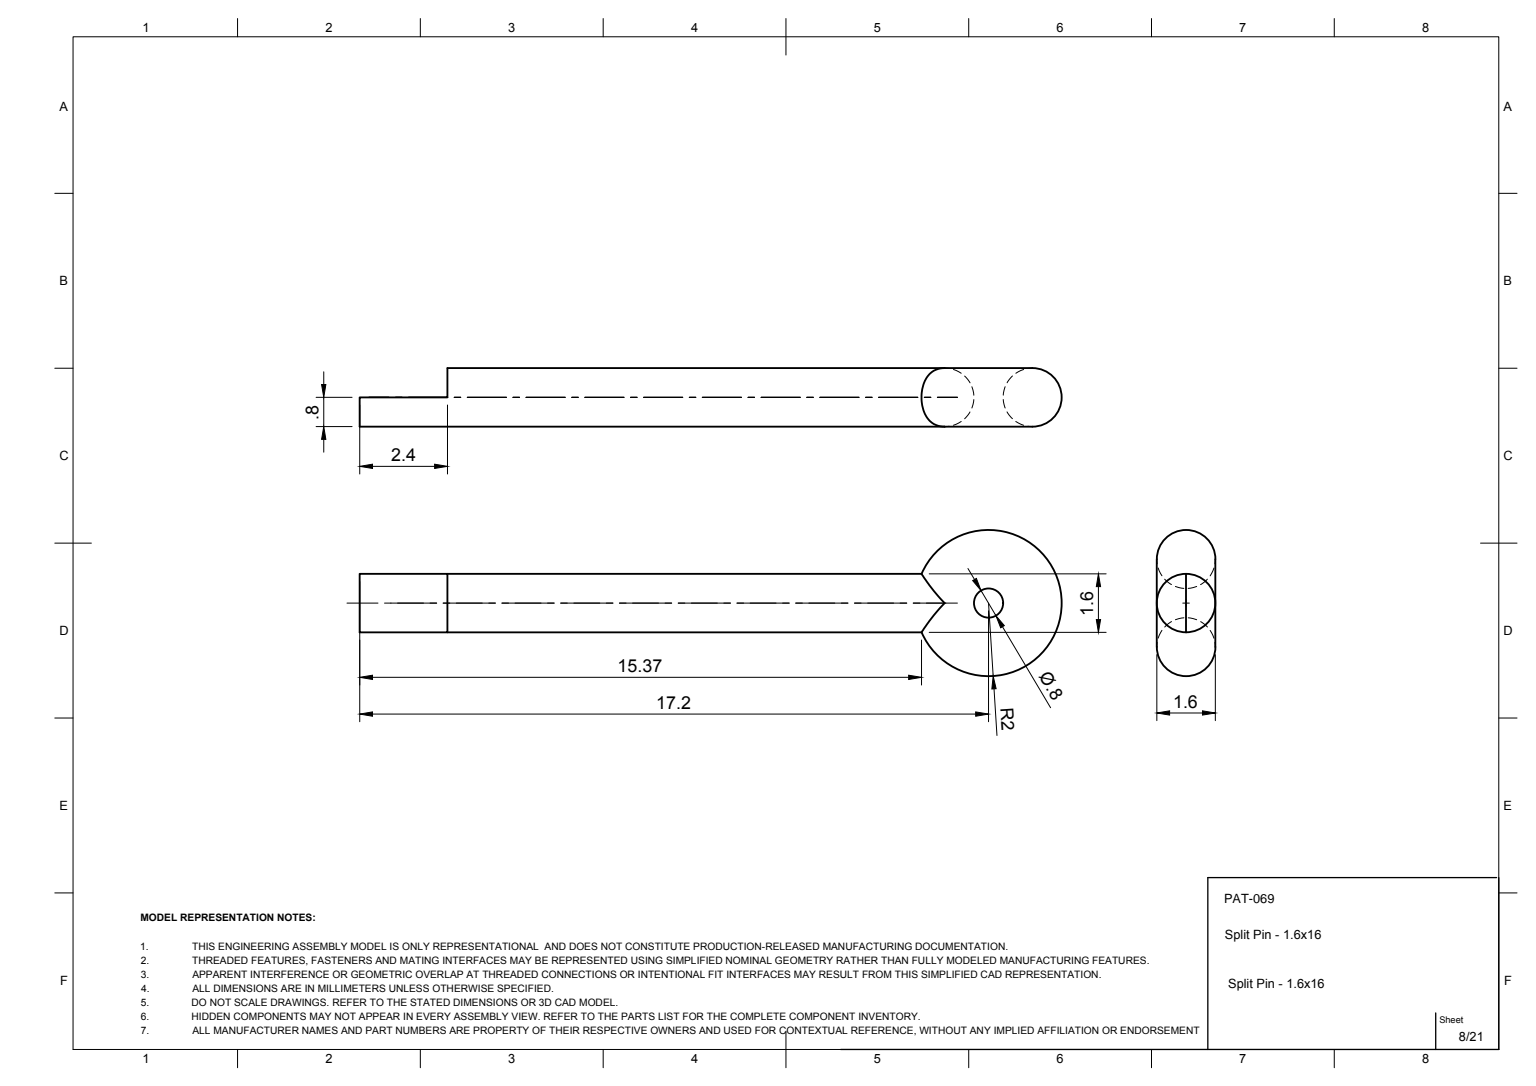
ISO-10303-21;
HEADER;
/* Generated by software containing ST-Developer
 * from STEP Tools, Inc. (www.steptools.com) 
 */

FILE_DESCRIPTION(
/* description */ ('Located fixture plate with toggle clamp'),
/* implementation_level */ '2;1');

FILE_NAME(
/* name */ 'Split Pin - 1.6x16.step',
/* time_stamp */ '2026-10-27T21:36:12-07:00',
/* author */ (''),
/* organization */ (''),
/* preprocessor_version */ 'ST-DEVELOPER v20.2',
/* originating_system */ 'Autodesk Translation Framework v15.17.0.0',
/* authorisation */ '');

FILE_SCHEMA (('AUTOMOTIVE_DESIGN { 1 0 10303 214 3 1 1 }'));
ENDSEC;

DATA;
#10=MECHANICAL_DESIGN_GEOMETRIC_PRESENTATION_REPRESENTATION('',(#344),#9285);
#11=TOROIDAL_SURFACE('',#5974,0.12,0.08);
#16=B_SPLINE_CURVE_WITH_KNOTS('',3,(#9112,#9113,#9114,#9115,#9116,#9117,
#9118,#9119,#9120,#9121,#9122,#9123,#9124,#9125,#9126,#9127,#9128,#9129,
#9130,#9131,#9132,#9133,#9134,#9135,#9136,#9137),.UNSPECIFIED.,.F.,.F.,
(4,2,2,2,2,2,2,2,2,2,2,2,4),(-0.00054581412719389,0.,0.0281583564005144,
0.0618496465371181,0.0905865724114538,0.120694112793616,0.144966158459363,
0.16923820412511,0.199345744507272,0.228082670381608,0.261773960518212,
0.289932316918681,0.290478131045882),.UNSPECIFIED.);
#17=B_SPLINE_CURVE_WITH_KNOTS('',3,(#9138,#9139,#9140,#9141,#9142,#9143,
#9144,#9145,#9146,#9147,#9148,#9149,#9150,#9151,#9152,#9153,#9154,#9155,
#9156,#9157,#9158,#9159,#9160,#9161,#9162,#9163),.UNSPECIFIED.,.F.,.F.,
(4,2,2,2,2,2,2,2,2,2,2,2,4),(-0.000545814127196571,0.,0.0281583564006391,
0.0618496465374156,0.0905865724118984,0.120694112794215,0.144966158460086,
0.169238204125958,0.199345744508275,0.228082670382758,0.261773960519534,
0.289932316920171,0.29047813104737),.UNSPECIFIED.);
#296=SHAPE_REPRESENTATION_RELATIONSHIP('SRR','None',#9422,#320);
#320=ADVANCED_BREP_SHAPE_REPRESENTATION('',(#365),#9284);
#344=STYLED_ITEM('',(#9612),#365);
#365=MANIFOLD_SOLID_BREP('Body1',#5195);
#485=FACE_BOUND('',#1378,.T.);
#670=PLANE('',#5977);
#671=PLANE('',#5979);
#672=PLANE('',#5983);
#963=FACE_OUTER_BOUND('',#1377,.T.);
#964=FACE_OUTER_BOUND('',#1379,.T.);
#965=FACE_OUTER_BOUND('',#1380,.T.);
#966=FACE_OUTER_BOUND('',#1381,.T.);
#967=FACE_OUTER_BOUND('',#1382,.T.);
#1377=EDGE_LOOP('',(#4768,#4769,#4770,#4771));
#1378=EDGE_LOOP('',(#4772,#4773));
#1379=EDGE_LOOP('',(#4774,#4775));
#1380=EDGE_LOOP('',(#4776,#4777,#4778,#4779));
#1381=EDGE_LOOP('',(#4780,#4781,#4782,#4783,#4784,#4785,#4786,#4787,#4788));
#1382=EDGE_LOOP('',(#4789,#4790,#4791));
#1576=CIRCLE('',#5975,0.08);
#1577=CIRCLE('',#5976,0.04);
#1578=CIRCLE('',#5978,0.08);
#1579=CIRCLE('',#5981,0.08);
#1580=CIRCLE('',#5982,0.08);
#1986=LINE('',#9168,#2396);
#1987=LINE('',#9171,#2397);
#1988=LINE('',#9173,#2398);
#1989=LINE('',#9174,#2399);
#1990=LINE('',#9178,#2400);
#2396=VECTOR('',#7470,1.);
#2397=VECTOR('',#7473,1.);
#2398=VECTOR('',#7474,1.);
#2399=VECTOR('',#7475,1.);
#2400=VECTOR('',#7480,0.08);
#2822=VERTEX_POINT('',#9107);
#2823=VERTEX_POINT('',#9110);
#2824=VERTEX_POINT('',#9111);
#2825=VERTEX_POINT('',#9165);
#2826=VERTEX_POINT('',#9166);
#2827=VERTEX_POINT('',#9170);
#2828=VERTEX_POINT('',#9172);
#2829=VERTEX_POINT('',#9176);
#3472=EDGE_CURVE('',#2822,#2822,#1576,.T.);
#3473=EDGE_CURVE('',#2822,#2822,#1577,.T.);
#3474=EDGE_CURVE('',#2823,#2824,#16,.T.);
#3475=EDGE_CURVE('',#2824,#2823,#17,.T.);
#3476=EDGE_CURVE('',#2825,#2826,#1578,.T.);
#3477=EDGE_CURVE('',#2825,#2826,#1986,.T.);
#3478=EDGE_CURVE('',#2826,#2827,#1987,.T.);
#3479=EDGE_CURVE('',#2828,#2827,#1988,.T.);
#3480=EDGE_CURVE('',#2825,#2828,#1989,.T.);
#3481=EDGE_CURVE('',#2829,#2828,#1579,.T.);
#3482=EDGE_CURVE('',#2829,#2824,#1990,.T.);
#3483=EDGE_CURVE('',#2827,#2829,#1580,.T.);
#4768=ORIENTED_EDGE('',*,*,#3472,.F.);
#4769=ORIENTED_EDGE('',*,*,#3473,.T.);
#4770=ORIENTED_EDGE('',*,*,#3472,.T.);
#4771=ORIENTED_EDGE('',*,*,#3473,.F.);
#4772=ORIENTED_EDGE('',*,*,#3474,.F.);
#4773=ORIENTED_EDGE('',*,*,#3475,.F.);
#4774=ORIENTED_EDGE('',*,*,#3476,.T.);
#4775=ORIENTED_EDGE('',*,*,#3477,.F.);
#4776=ORIENTED_EDGE('',*,*,#3477,.T.);
#4777=ORIENTED_EDGE('',*,*,#3478,.T.);
#4778=ORIENTED_EDGE('',*,*,#3479,.F.);
#4779=ORIENTED_EDGE('',*,*,#3480,.F.);
#4780=ORIENTED_EDGE('',*,*,#3476,.F.);
#4781=ORIENTED_EDGE('',*,*,#3480,.T.);
#4782=ORIENTED_EDGE('',*,*,#3481,.F.);
#4783=ORIENTED_EDGE('',*,*,#3482,.T.);
#4784=ORIENTED_EDGE('',*,*,#3475,.T.);
#4785=ORIENTED_EDGE('',*,*,#3474,.T.);
#4786=ORIENTED_EDGE('',*,*,#3482,.F.);
#4787=ORIENTED_EDGE('',*,*,#3483,.F.);
#4788=ORIENTED_EDGE('',*,*,#3478,.F.);
#4789=ORIENTED_EDGE('',*,*,#3483,.T.);
#4790=ORIENTED_EDGE('',*,*,#3481,.T.);
#4791=ORIENTED_EDGE('',*,*,#3479,.T.);
#4873=CYLINDRICAL_SURFACE('',#5980,0.08);
#5164=ADVANCED_FACE('',(#963,#485),#11,.T.);
#5165=ADVANCED_FACE('',(#964),#670,.F.);
#5166=ADVANCED_FACE('',(#965),#671,.T.);
#5167=ADVANCED_FACE('',(#966),#4873,.T.);
#5168=ADVANCED_FACE('',(#967),#672,.F.);
#5195=CLOSED_SHELL('',(#5164,#5165,#5166,#5167,#5168));
#5973=AXIS2_PLACEMENT_3D('',#9105,#7458,#7459);
#5974=AXIS2_PLACEMENT_3D('',#9106,#7460,#7461);
#5975=AXIS2_PLACEMENT_3D('',#9108,#7462,#7463);
#5976=AXIS2_PLACEMENT_3D('',#9109,#7464,#7465);
#5977=AXIS2_PLACEMENT_3D('',#9164,#7466,#7467);
#5978=AXIS2_PLACEMENT_3D('',#9167,#7468,#7469);
#5979=AXIS2_PLACEMENT_3D('',#9169,#7471,#7472);
#5980=AXIS2_PLACEMENT_3D('',#9175,#7476,#7477);
#5981=AXIS2_PLACEMENT_3D('',#9177,#7478,#7479);
#5982=AXIS2_PLACEMENT_3D('',#9179,#7481,#7482);
#5983=AXIS2_PLACEMENT_3D('',#9180,#7483,#7484);
#7458=DIRECTION('axis',(0.,0.,1.));
#7459=DIRECTION('refdir',(1.,0.,0.));
#7460=DIRECTION('center_axis',(-1.,0.,0.));
#7461=DIRECTION('ref_axis',(0.,0.,1.));
#7462=DIRECTION('center_axis',(0.,-1.,1.38777878078145E-16));
#7463=DIRECTION('ref_axis',(0.,-1.38777878078145E-16,-1.));
#7464=DIRECTION('center_axis',(1.,0.,0.));
#7465=DIRECTION('ref_axis',(0.,0.,1.));
#7466=DIRECTION('center_axis',(0.,1.,0.));
#7467=DIRECTION('ref_axis',(1.,0.,0.));
#7468=DIRECTION('center_axis',(0.,-1.,0.));
#7469=DIRECTION('ref_axis',(1.,0.,0.));
#7470=DIRECTION('',(0.,0.,1.));
#7471=DIRECTION('center_axis',(1.,0.,0.));
#7472=DIRECTION('ref_axis',(0.,0.,1.));
#7473=DIRECTION('',(0.,-1.,0.));
#7474=DIRECTION('',(0.,0.,1.));
#7475=DIRECTION('',(0.,-1.,0.));
#7476=DIRECTION('center_axis',(0.,-1.,0.));
#7477=DIRECTION('ref_axis',(1.,0.,0.));
#7478=DIRECTION('center_axis',(0.,-1.,0.));
#7479=DIRECTION('ref_axis',(1.,0.,0.));
#7480=DIRECTION('',(0.,1.,0.));
#7481=DIRECTION('center_axis',(0.,-1.,0.));
#7482=DIRECTION('ref_axis',(1.,0.,0.));
#7483=DIRECTION('center_axis',(0.,1.,0.));
#7484=DIRECTION('ref_axis',(1.,0.,0.));
#9105=CARTESIAN_POINT('',(0.,0.,0.));
#9106=CARTESIAN_POINT('Origin',(0.,0.12,0.));
#9107=CARTESIAN_POINT('',(-9.79717439317883E-18,0.12,-0.04));
#9108=CARTESIAN_POINT('Origin',(0.,0.12,-0.12));
#9109=CARTESIAN_POINT('Origin',(9.79717439317883E-18,0.12,0.));
#9110=CARTESIAN_POINT('',(0.08,-4.89858719658941E-18,7.34788079488412E-18));
#9111=CARTESIAN_POINT('',(-0.08,-4.89858719658941E-18,7.34788079488412E-18));
#9112=CARTESIAN_POINT('Ctrl Pts',(0.08,-4.89858719658941E-18,7.34788079488412E-18));
#9113=CARTESIAN_POINT('Ctrl Pts',(0.08,-0.00012864962353541,0.000128649623535413));
#9114=CARTESIAN_POINT('Ctrl Pts',(0.0799996896739287,-0.00025719571182076,
0.000257402596003253));
#9115=CARTESIAN_POINT('Ctrl Pts',(0.0799669711262291,-0.00701193164572964,
0.00703384588894362));
#9116=CARTESIAN_POINT('Ctrl Pts',(0.0791054994909294,-0.0133457972655825,
0.0139383126556792));
#9117=CARTESIAN_POINT('Ctrl Pts',(0.0749700088488058,-0.0265076530862524,
0.0292212026164895));
#9118=CARTESIAN_POINT('Ctrl Pts',(0.0712702072865517,-0.0331317062461458,
0.0375603420117568));
#9119=CARTESIAN_POINT('Ctrl Pts',(0.0612858949407667,-0.0440683985740427,
0.0520545604187517));
#9120=CARTESIAN_POINT('Ctrl Pts',(0.0555090276731744,-0.0485199197794574,
0.0582717815295611));
#9121=CARTESIAN_POINT('Ctrl Pts',(0.0412398082144208,-0.0561090538733877,
0.0691638397919718));
#9122=CARTESIAN_POINT('Ctrl Pts',(0.0327878980890048,-0.059089642483296,
0.0736229049587921));
#9123=CARTESIAN_POINT('Ctrl Pts',(0.0159233027310102,-0.0625179833270725,
0.0787936360751706));
#9124=CARTESIAN_POINT('Ctrl Pts',(0.00801661414593076,-0.0633030277982336,
0.08));
#9125=CARTESIAN_POINT('Ctrl Pts',(-0.00801661414593074,-0.0633030277982336,
0.08));
#9126=CARTESIAN_POINT('Ctrl Pts',(-0.0159233027310102,-0.0625179833270726,
0.0787936360751706));
#9127=CARTESIAN_POINT('Ctrl Pts',(-0.0327878980890049,-0.059089642483296,
0.0736229049587921));
#9128=CARTESIAN_POINT('Ctrl Pts',(-0.0412398082144209,-0.0561090538733877,
0.0691638397919717));
#9129=CARTESIAN_POINT('Ctrl Pts',(-0.0555090276731744,-0.0485199197794574,
0.0582717815295611));
#9130=CARTESIAN_POINT('Ctrl Pts',(-0.0612858949407667,-0.0440683985740427,
0.0520545604187517));
#9131=CARTESIAN_POINT('Ctrl Pts',(-0.0712702072865517,-0.0331317062461458,
0.0375603420117568));
#9132=CARTESIAN_POINT('Ctrl Pts',(-0.0749700088488058,-0.0265076530862524,
0.0292212026164895));
#9133=CARTESIAN_POINT('Ctrl Pts',(-0.0791054994909264,-0.0133457972655921,
0.0139383126556903));
#9134=CARTESIAN_POINT('Ctrl Pts',(-0.0799669711262287,-0.00701193164579759,
0.0070338458890125));
#9135=CARTESIAN_POINT('Ctrl Pts',(-0.0799996896739287,-0.000257195711817665,
0.000257402596000083));
#9136=CARTESIAN_POINT('Ctrl Pts',(-0.08,-0.000128649623538514,0.000128649623538516));
#9137=CARTESIAN_POINT('Ctrl Pts',(-0.08,-4.89858719658941E-18,7.34788079488412E-18));
#9138=CARTESIAN_POINT('Ctrl Pts',(-0.08,-4.89858719658941E-18,7.34788079488412E-18));
#9139=CARTESIAN_POINT('Ctrl Pts',(-0.08,-0.000128649623536042,-0.00012864962353603));
#9140=CARTESIAN_POINT('Ctrl Pts',(-0.0799996896739287,-0.000257195711820127,
-0.000257402596002604));
#9141=CARTESIAN_POINT('Ctrl Pts',(-0.0799669711262289,-0.0070119316457589,
-0.00703384588897312));
#9142=CARTESIAN_POINT('Ctrl Pts',(-0.0791054994909281,-0.0133457972655867,
-0.0139383126556841));
#9143=CARTESIAN_POINT('Ctrl Pts',(-0.0749700088488058,-0.0265076530862525,
-0.0292212026164896));
#9144=CARTESIAN_POINT('Ctrl Pts',(-0.0712702072865516,-0.0331317062461459,
-0.0375603420117568));
#9145=CARTESIAN_POINT('Ctrl Pts',(-0.0612858949407667,-0.0440683985740427,
-0.0520545604187517));
#9146=CARTESIAN_POINT('Ctrl Pts',(-0.0555090276731744,-0.0485199197794574,
-0.0582717815295611));
#9147=CARTESIAN_POINT('Ctrl Pts',(-0.0412398082144209,-0.0561090538733877,
-0.0691638397919717));
#9148=CARTESIAN_POINT('Ctrl Pts',(-0.0327878980890049,-0.059089642483296,
-0.0736229049587921));
#9149=CARTESIAN_POINT('Ctrl Pts',(-0.0159233027310101,-0.0625179833270725,
-0.0787936360751706));
#9150=CARTESIAN_POINT('Ctrl Pts',(-0.00801661414593069,-0.0633030277982336,
-0.08));
#9151=CARTESIAN_POINT('Ctrl Pts',(0.0080166141459307,-0.0633030277982336,
-0.08));
#9152=CARTESIAN_POINT('Ctrl Pts',(0.0159233027310101,-0.0625179833270725,
-0.0787936360751706));
#9153=CARTESIAN_POINT('Ctrl Pts',(0.0327878980890049,-0.0590896424832959,
-0.0736229049587921));
#9154=CARTESIAN_POINT('Ctrl Pts',(0.0412398082144209,-0.0561090538733877,
-0.0691638397919717));
#9155=CARTESIAN_POINT('Ctrl Pts',(0.0555090276731744,-0.0485199197794574,
-0.0582717815295611));
#9156=CARTESIAN_POINT('Ctrl Pts',(0.0612858949407666,-0.0440683985740428,
-0.0520545604187518));
#9157=CARTESIAN_POINT('Ctrl Pts',(0.0712702072865517,-0.0331317062461458,
-0.0375603420117568));
#9158=CARTESIAN_POINT('Ctrl Pts',(0.0749700088488058,-0.0265076530862524,
-0.0292212026164895));
#9159=CARTESIAN_POINT('Ctrl Pts',(0.079105499490928,-0.013345797265587,
-0.0139383126556845));
#9160=CARTESIAN_POINT('Ctrl Pts',(0.0799669711262289,-0.00701193164576148,
-0.00703384588897579));
#9161=CARTESIAN_POINT('Ctrl Pts',(0.0799996896739287,-0.000257195711819584,
-0.000257402596002039));
#9162=CARTESIAN_POINT('Ctrl Pts',(0.08,-0.000128649623536605,-0.000128649623536593));
#9163=CARTESIAN_POINT('Ctrl Pts',(0.08,-4.89858719658941E-18,7.34788079488412E-18));
#9164=CARTESIAN_POINT('Origin',(0.04,-1.36,0.));
#9165=CARTESIAN_POINT('',(0.,-1.36,-0.08));
#9166=CARTESIAN_POINT('',(0.,-1.36,0.08));
#9167=CARTESIAN_POINT('Origin',(0.,-1.36,0.));
#9168=CARTESIAN_POINT('',(0.,-1.36,-0.04));
#9169=CARTESIAN_POINT('Origin',(0.,0.,-0.08));
#9170=CARTESIAN_POINT('',(0.,-1.6,0.08));
#9171=CARTESIAN_POINT('',(0.,0.,0.08));
#9172=CARTESIAN_POINT('',(0.,-1.6,-0.08));
#9173=CARTESIAN_POINT('',(0.,-1.6,-0.09));
#9174=CARTESIAN_POINT('',(0.,0.,-0.08));
#9175=CARTESIAN_POINT('Origin',(0.,0.,0.));
#9176=CARTESIAN_POINT('',(-0.08,-1.6,-9.79717439317883E-18));
#9177=CARTESIAN_POINT('Origin',(0.,-1.6,0.));
#9178=CARTESIAN_POINT('',(-0.08,0.,-9.79717439317883E-18));
#9179=CARTESIAN_POINT('Origin',(0.,-1.6,0.));
#9180=CARTESIAN_POINT('Origin',(-0.04,-1.6,0.));
#9254=UNCERTAINTY_MEASURE_WITH_UNIT(LENGTH_MEASURE(0.001),#9286,
'DISTANCE_ACCURACY_VALUE',
'Maximum model space distance between geometric entities at asserted c
onnectivities');
#9255=UNCERTAINTY_MEASURE_WITH_UNIT(LENGTH_MEASURE(0.001),#9286,
'DISTANCE_ACCURACY_VALUE',
'Maximum model space distance between geometric entities at asserted c
onnectivities');
#9284=(
GEOMETRIC_REPRESENTATION_CONTEXT(3)
GLOBAL_UNCERTAINTY_ASSIGNED_CONTEXT((#9254))
GLOBAL_UNIT_ASSIGNED_CONTEXT((#9286,#9288,#9289))
REPRESENTATION_CONTEXT('','3D')
);
#9285=(
GEOMETRIC_REPRESENTATION_CONTEXT(3)
GLOBAL_UNCERTAINTY_ASSIGNED_CONTEXT((#9255))
GLOBAL_UNIT_ASSIGNED_CONTEXT((#9286,#9288,#9289))
REPRESENTATION_CONTEXT('','3D')
);
#9286=(
LENGTH_UNIT()
NAMED_UNIT(*)
SI_UNIT(.CENTI.,.METRE.)
);
#9288=(
NAMED_UNIT(*)
PLANE_ANGLE_UNIT()
SI_UNIT($,.RADIAN.)
);
#9289=(
NAMED_UNIT(*)
SI_UNIT($,.STERADIAN.)
SOLID_ANGLE_UNIT()
);
#9318=SHAPE_DEFINITION_REPRESENTATION(#9348,#9422);
#9348=PRODUCT_DEFINITION_SHAPE('',$,#9452);
#9422=SHAPE_REPRESENTATION('',(#5973),#9284);
#9423=PRODUCT_DEFINITION_CONTEXT('part definition',#9512,'design');
#9452=PRODUCT_DEFINITION('Split Pin - 1.6x16','Split Pin - 1.6x16',#9481,
#9423);
#9481=PRODUCT_DEFINITION_FORMATION('',$,#9542);
#9512=APPLICATION_CONTEXT(
'Core Data for Automotive Mechanical Design Process');
#9513=PRODUCT_CONTEXT('part definition',#9512,'mechanical');
#9542=PRODUCT('Split Pin - 1.6x16','Split Pin - 1.6x16',
'Split Pin - 1.6x16',(#9513));
#9606=COLOUR_RGB('Grey',0.48,0.52,0.57);
#9607=FILL_AREA_STYLE_COLOUR('',#9606);
#9608=FILL_AREA_STYLE('',(#9607));
#9609=SURFACE_STYLE_FILL_AREA(#9608);
#9610=SURFACE_SIDE_STYLE('',(#9609));
#9611=SURFACE_STYLE_USAGE(.BOTH.,#9610);
#9612=PRESENTATION_STYLE_ASSIGNMENT((#9611));
ENDSEC;
END-ISO-10303-21;
